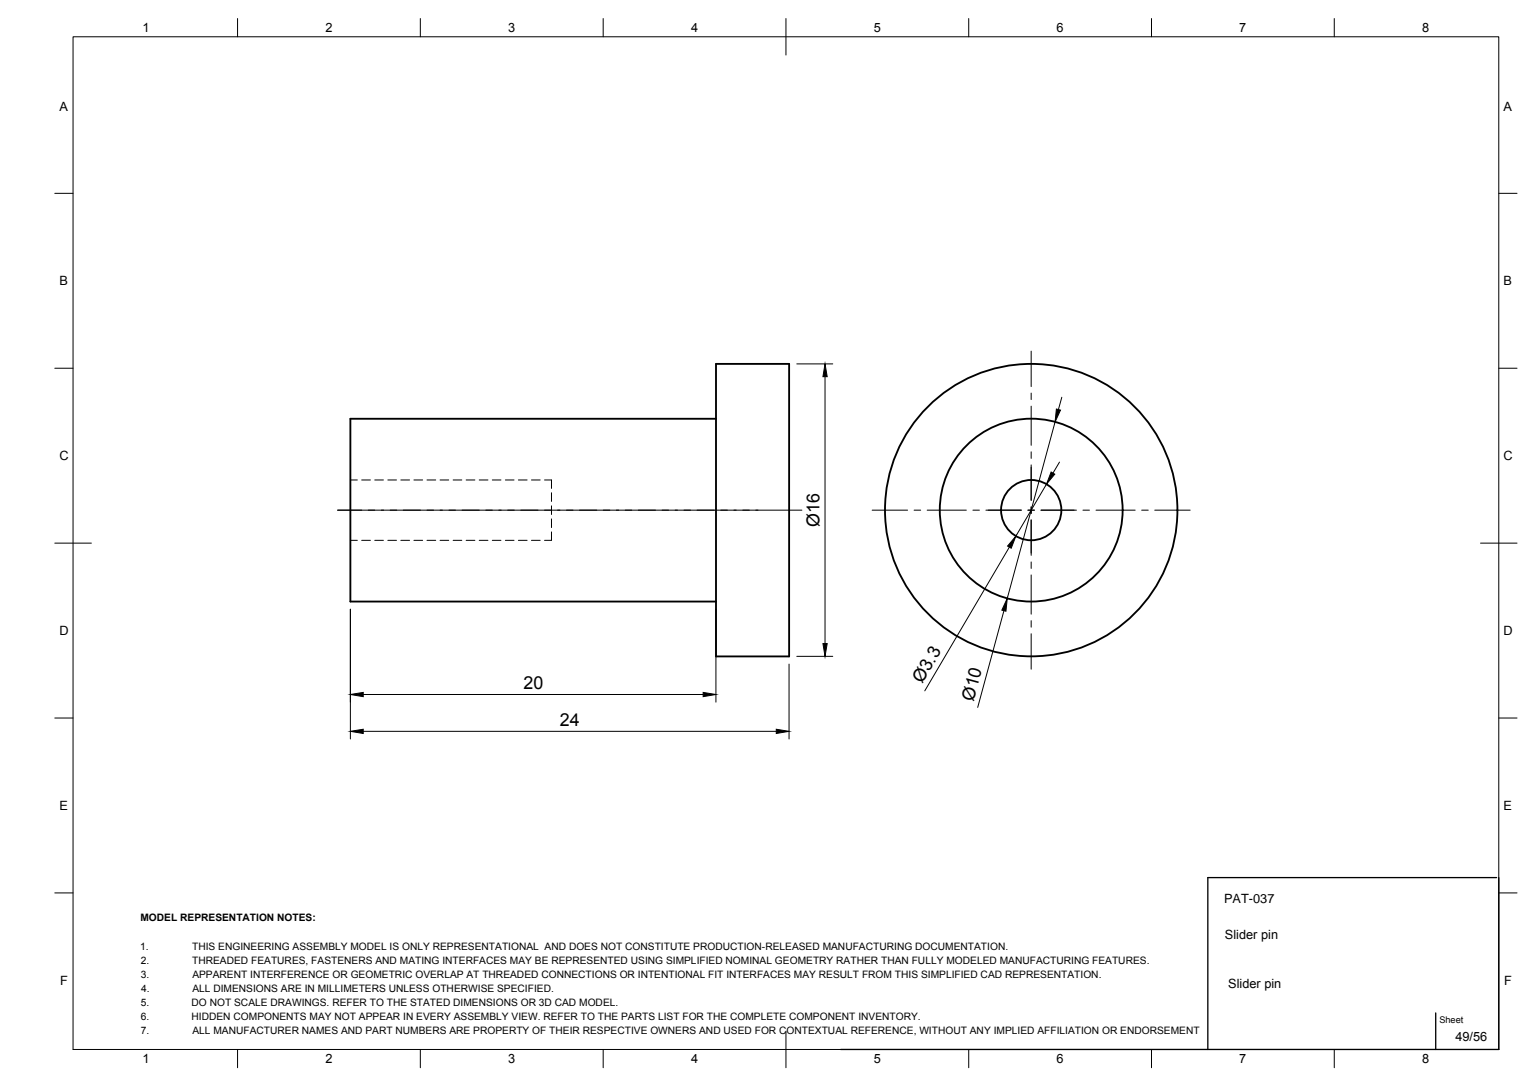
ISO-10303-21;
HEADER;
/* Generated by software containing ST-Developer
 * from STEP Tools, Inc. (www.steptools.com) 
 */

FILE_DESCRIPTION(
/* description */ ('Flywheel Crank-Slider'),
/* implementation_level */ '2;1');

FILE_NAME(
/* name */ 'Slider pin.step',
/* time_stamp */ '2026-10-28T03:23:13-07:00',
/* author */ (''),
/* organization */ (''),
/* preprocessor_version */ 'ST-DEVELOPER v20.2',
/* originating_system */ 'Autodesk Translation Framework v15.17.0.0',
/* authorisation */ '');

FILE_SCHEMA (('AUTOMOTIVE_DESIGN { 1 0 10303 214 3 1 1 }'));
ENDSEC;

DATA;
#10=MECHANICAL_DESIGN_GEOMETRIC_PRESENTATION_REPRESENTATION('',(#722),#17322);
#609=SHAPE_REPRESENTATION_RELATIONSHIP('SRR','None',#17610,#661);
#661=ADVANCED_BREP_SHAPE_REPRESENTATION('',(#779),#17314);
#722=STYLED_ITEM('',(#17931),#779);
#779=MANIFOLD_SOLID_BREP('Body1',#9104);
#991=FACE_BOUND('',#2539,.T.);
#992=FACE_BOUND('',#2544,.T.);
#1282=PLANE('',#10622);
#1283=PLANE('',#10623);
#1284=PLANE('',#10628);
#1285=PLANE('',#10631);
#1795=FACE_OUTER_BOUND('',#2536,.T.);
#1796=FACE_OUTER_BOUND('',#2537,.T.);
#1797=FACE_OUTER_BOUND('',#2538,.T.);
#1798=FACE_OUTER_BOUND('',#2540,.T.);
#1799=FACE_OUTER_BOUND('',#2541,.T.);
#1800=FACE_OUTER_BOUND('',#2542,.T.);
#1801=FACE_OUTER_BOUND('',#2543,.T.);
#2536=EDGE_LOOP('',(#8120,#8121,#8122,#8123));
#2537=EDGE_LOOP('',(#8124));
#2538=EDGE_LOOP('',(#8125));
#2539=EDGE_LOOP('',(#8126));
#2540=EDGE_LOOP('',(#8127,#8128,#8129,#8130));
#2541=EDGE_LOOP('',(#8131));
#2542=EDGE_LOOP('',(#8132,#8133,#8134,#8135));
#2543=EDGE_LOOP('',(#8136));
#2544=EDGE_LOOP('',(#8137));
#3169=LINE('',#16867,#3780);
#3170=LINE('',#16877,#3781);
#3171=LINE('',#16883,#3782);
#3780=VECTOR('',#13255,0.164999999999999);
#3781=VECTOR('',#13268,0.800000000000001);
#3782=VECTOR('',#13277,0.5);
#4230=CIRCLE('',#10620,0.164999999999999);
#4231=CIRCLE('',#10621,0.164999999999999);
#4232=CIRCLE('',#10624,0.800000000000001);
#4233=CIRCLE('',#10625,0.5);
#4234=CIRCLE('',#10627,0.800000000000001);
#4235=CIRCLE('',#10630,0.5);
#4949=VERTEX_POINT('',#16864);
#4950=VERTEX_POINT('',#16866);
#4951=VERTEX_POINT('',#16871);
#4952=VERTEX_POINT('',#16873);
#4953=VERTEX_POINT('',#16876);
#4954=VERTEX_POINT('',#16881);
#6017=EDGE_CURVE('',#4949,#4949,#4230,.T.);
#6018=EDGE_CURVE('',#4949,#4950,#3169,.T.);
#6019=EDGE_CURVE('',#4950,#4950,#4231,.T.);
#6020=EDGE_CURVE('',#4951,#4951,#4232,.T.);
#6021=EDGE_CURVE('',#4952,#4952,#4233,.T.);
#6022=EDGE_CURVE('',#4951,#4953,#3170,.T.);
#6023=EDGE_CURVE('',#4953,#4953,#4234,.T.);
#6024=EDGE_CURVE('',#4954,#4954,#4235,.T.);
#6025=EDGE_CURVE('',#4954,#4952,#3171,.T.);
#8120=ORIENTED_EDGE('',*,*,#6017,.F.);
#8121=ORIENTED_EDGE('',*,*,#6018,.T.);
#8122=ORIENTED_EDGE('',*,*,#6019,.F.);
#8123=ORIENTED_EDGE('',*,*,#6018,.F.);
#8124=ORIENTED_EDGE('',*,*,#6017,.T.);
#8125=ORIENTED_EDGE('',*,*,#6020,.T.);
#8126=ORIENTED_EDGE('',*,*,#6021,.F.);
#8127=ORIENTED_EDGE('',*,*,#6020,.F.);
#8128=ORIENTED_EDGE('',*,*,#6022,.T.);
#8129=ORIENTED_EDGE('',*,*,#6023,.T.);
#8130=ORIENTED_EDGE('',*,*,#6022,.F.);
#8131=ORIENTED_EDGE('',*,*,#6023,.F.);
#8132=ORIENTED_EDGE('',*,*,#6024,.F.);
#8133=ORIENTED_EDGE('',*,*,#6025,.T.);
#8134=ORIENTED_EDGE('',*,*,#6021,.T.);
#8135=ORIENTED_EDGE('',*,*,#6025,.F.);
#8136=ORIENTED_EDGE('',*,*,#6024,.T.);
#8137=ORIENTED_EDGE('',*,*,#6019,.T.);
#8492=CYLINDRICAL_SURFACE('',#10619,0.164999999999999);
#8493=CYLINDRICAL_SURFACE('',#10626,0.800000000000001);
#8494=CYLINDRICAL_SURFACE('',#10629,0.5);
#8986=ADVANCED_FACE('',(#1795),#8492,.F.);
#8987=ADVANCED_FACE('',(#1796),#1282,.T.);
#8988=ADVANCED_FACE('',(#1797,#991),#1283,.T.);
#8989=ADVANCED_FACE('',(#1798),#8493,.T.);
#8990=ADVANCED_FACE('',(#1799),#1284,.F.);
#8991=ADVANCED_FACE('',(#1800),#8494,.T.);
#8992=ADVANCED_FACE('',(#1801,#992),#1285,.T.);
#9104=CLOSED_SHELL('',(#8986,#8987,#8988,#8989,#8990,#8991,#8992));
#10618=AXIS2_PLACEMENT_3D('',#16862,#13249,#13250);
#10619=AXIS2_PLACEMENT_3D('',#16863,#13251,#13252);
#10620=AXIS2_PLACEMENT_3D('',#16865,#13253,#13254);
#10621=AXIS2_PLACEMENT_3D('',#16868,#13256,#13257);
#10622=AXIS2_PLACEMENT_3D('',#16869,#13258,#13259);
#10623=AXIS2_PLACEMENT_3D('',#16870,#13260,#13261);
#10624=AXIS2_PLACEMENT_3D('',#16872,#13262,#13263);
#10625=AXIS2_PLACEMENT_3D('',#16874,#13264,#13265);
#10626=AXIS2_PLACEMENT_3D('',#16875,#13266,#13267);
#10627=AXIS2_PLACEMENT_3D('',#16878,#13269,#13270);
#10628=AXIS2_PLACEMENT_3D('',#16879,#13271,#13272);
#10629=AXIS2_PLACEMENT_3D('',#16880,#13273,#13274);
#10630=AXIS2_PLACEMENT_3D('',#16882,#13275,#13276);
#10631=AXIS2_PLACEMENT_3D('',#16884,#13278,#13279);
#13249=DIRECTION('axis',(0.,0.,1.));
#13250=DIRECTION('refdir',(1.,0.,0.));
#13251=DIRECTION('center_axis',(0.,1.,0.));
#13252=DIRECTION('ref_axis',(1.,0.,0.));
#13253=DIRECTION('center_axis',(0.,1.,0.));
#13254=DIRECTION('ref_axis',(1.,0.,0.));
#13255=DIRECTION('',(0.,1.,0.));
#13256=DIRECTION('center_axis',(0.,-1.,0.));
#13257=DIRECTION('ref_axis',(1.,0.,0.));
#13258=DIRECTION('center_axis',(0.,1.,0.));
#13259=DIRECTION('ref_axis',(1.,0.,0.));
#13260=DIRECTION('center_axis',(0.,1.,0.));
#13261=DIRECTION('ref_axis',(1.,0.,0.));
#13262=DIRECTION('center_axis',(0.,1.,0.));
#13263=DIRECTION('ref_axis',(1.,0.,0.));
#13264=DIRECTION('center_axis',(0.,1.,0.));
#13265=DIRECTION('ref_axis',(1.,0.,0.));
#13266=DIRECTION('center_axis',(0.,1.,0.));
#13267=DIRECTION('ref_axis',(1.,0.,0.));
#13268=DIRECTION('',(0.,-1.,0.));
#13269=DIRECTION('center_axis',(0.,1.,0.));
#13270=DIRECTION('ref_axis',(1.,0.,0.));
#13271=DIRECTION('center_axis',(0.,1.,0.));
#13272=DIRECTION('ref_axis',(1.,0.,0.));
#13273=DIRECTION('center_axis',(0.,1.,0.));
#13274=DIRECTION('ref_axis',(1.,0.,0.));
#13275=DIRECTION('center_axis',(0.,1.,0.));
#13276=DIRECTION('ref_axis',(1.,0.,0.));
#13277=DIRECTION('',(0.,-1.,0.));
#13278=DIRECTION('center_axis',(0.,1.,0.));
#13279=DIRECTION('ref_axis',(1.,0.,0.));
#16862=CARTESIAN_POINT('',(0.,0.,0.));
#16863=CARTESIAN_POINT('Origin',(12.,2.7,10.));
#16864=CARTESIAN_POINT('',(11.835,2.7,10.));
#16865=CARTESIAN_POINT('Origin',(12.,2.7,10.));
#16866=CARTESIAN_POINT('',(11.835,3.8,10.));
#16867=CARTESIAN_POINT('',(11.835,2.7,10.));
#16868=CARTESIAN_POINT('Origin',(12.,3.8,10.));
#16869=CARTESIAN_POINT('Origin',(12.,2.7,10.));
#16870=CARTESIAN_POINT('Origin',(12.,1.8,10.));
#16871=CARTESIAN_POINT('',(11.2,1.8,10.));
#16872=CARTESIAN_POINT('Origin',(12.,1.8,10.));
#16873=CARTESIAN_POINT('',(11.5,1.8,10.));
#16874=CARTESIAN_POINT('Origin',(12.,1.8,10.));
#16875=CARTESIAN_POINT('Origin',(12.,1.4,10.));
#16876=CARTESIAN_POINT('',(11.2,1.4,10.));
#16877=CARTESIAN_POINT('',(11.2,1.4,10.));
#16878=CARTESIAN_POINT('Origin',(12.,1.4,10.));
#16879=CARTESIAN_POINT('Origin',(12.,1.4,10.));
#16880=CARTESIAN_POINT('Origin',(12.,1.8,10.));
#16881=CARTESIAN_POINT('',(11.5,3.8,10.));
#16882=CARTESIAN_POINT('Origin',(12.,3.8,10.));
#16883=CARTESIAN_POINT('',(11.5,1.8,10.));
#16884=CARTESIAN_POINT('Origin',(12.,3.8,10.));
#17253=UNCERTAINTY_MEASURE_WITH_UNIT(LENGTH_MEASURE(0.001),#17323,
'DISTANCE_ACCURACY_VALUE',
'Maximum model space distance between geometric entities at asserted c
onnectivities');
#17261=UNCERTAINTY_MEASURE_WITH_UNIT(LENGTH_MEASURE(0.001),#17323,
'DISTANCE_ACCURACY_VALUE',
'Maximum model space distance between geometric entities at asserted c
onnectivities');
#17314=(
GEOMETRIC_REPRESENTATION_CONTEXT(3)
GLOBAL_UNCERTAINTY_ASSIGNED_CONTEXT((#17253))
GLOBAL_UNIT_ASSIGNED_CONTEXT((#17323,#17325,#17326))
REPRESENTATION_CONTEXT('','3D')
);
#17322=(
GEOMETRIC_REPRESENTATION_CONTEXT(3)
GLOBAL_UNCERTAINTY_ASSIGNED_CONTEXT((#17261))
GLOBAL_UNIT_ASSIGNED_CONTEXT((#17323,#17325,#17326))
REPRESENTATION_CONTEXT('','3D')
);
#17323=(
LENGTH_UNIT()
NAMED_UNIT(*)
SI_UNIT(.CENTI.,.METRE.)
);
#17325=(
NAMED_UNIT(*)
PLANE_ANGLE_UNIT()
SI_UNIT($,.RADIAN.)
);
#17326=(
NAMED_UNIT(*)
SI_UNIT($,.STERADIAN.)
SOLID_ANGLE_UNIT()
);
#17379=SHAPE_DEFINITION_REPRESENTATION(#17453,#17610);
#17453=PRODUCT_DEFINITION_SHAPE('',$,#17671);
#17610=SHAPE_REPRESENTATION('',(#10618),#17314);
#17618=PRODUCT_DEFINITION_CONTEXT('part definition',#17800,'design');
#17671=PRODUCT_DEFINITION('Slider pin','Slider pin',#17731,#17618);
#17731=PRODUCT_DEFINITION_FORMATION('',$,#17854);
#17800=APPLICATION_CONTEXT(
'Core Data for Automotive Mechanical Design Process');
#17801=PRODUCT_CONTEXT('part definition',#17800,'mechanical');
#17854=PRODUCT('Slider pin','Slider pin','Slider pin',(#17801));
#17925=COLOUR_RGB('Grey',0.48,0.52,0.57);
#17926=FILL_AREA_STYLE_COLOUR('',#17925);
#17927=FILL_AREA_STYLE('',(#17926));
#17928=SURFACE_STYLE_FILL_AREA(#17927);
#17929=SURFACE_SIDE_STYLE('',(#17928));
#17930=SURFACE_STYLE_USAGE(.BOTH.,#17929);
#17931=PRESENTATION_STYLE_ASSIGNMENT((#17930));
ENDSEC;
END-ISO-10303-21;
